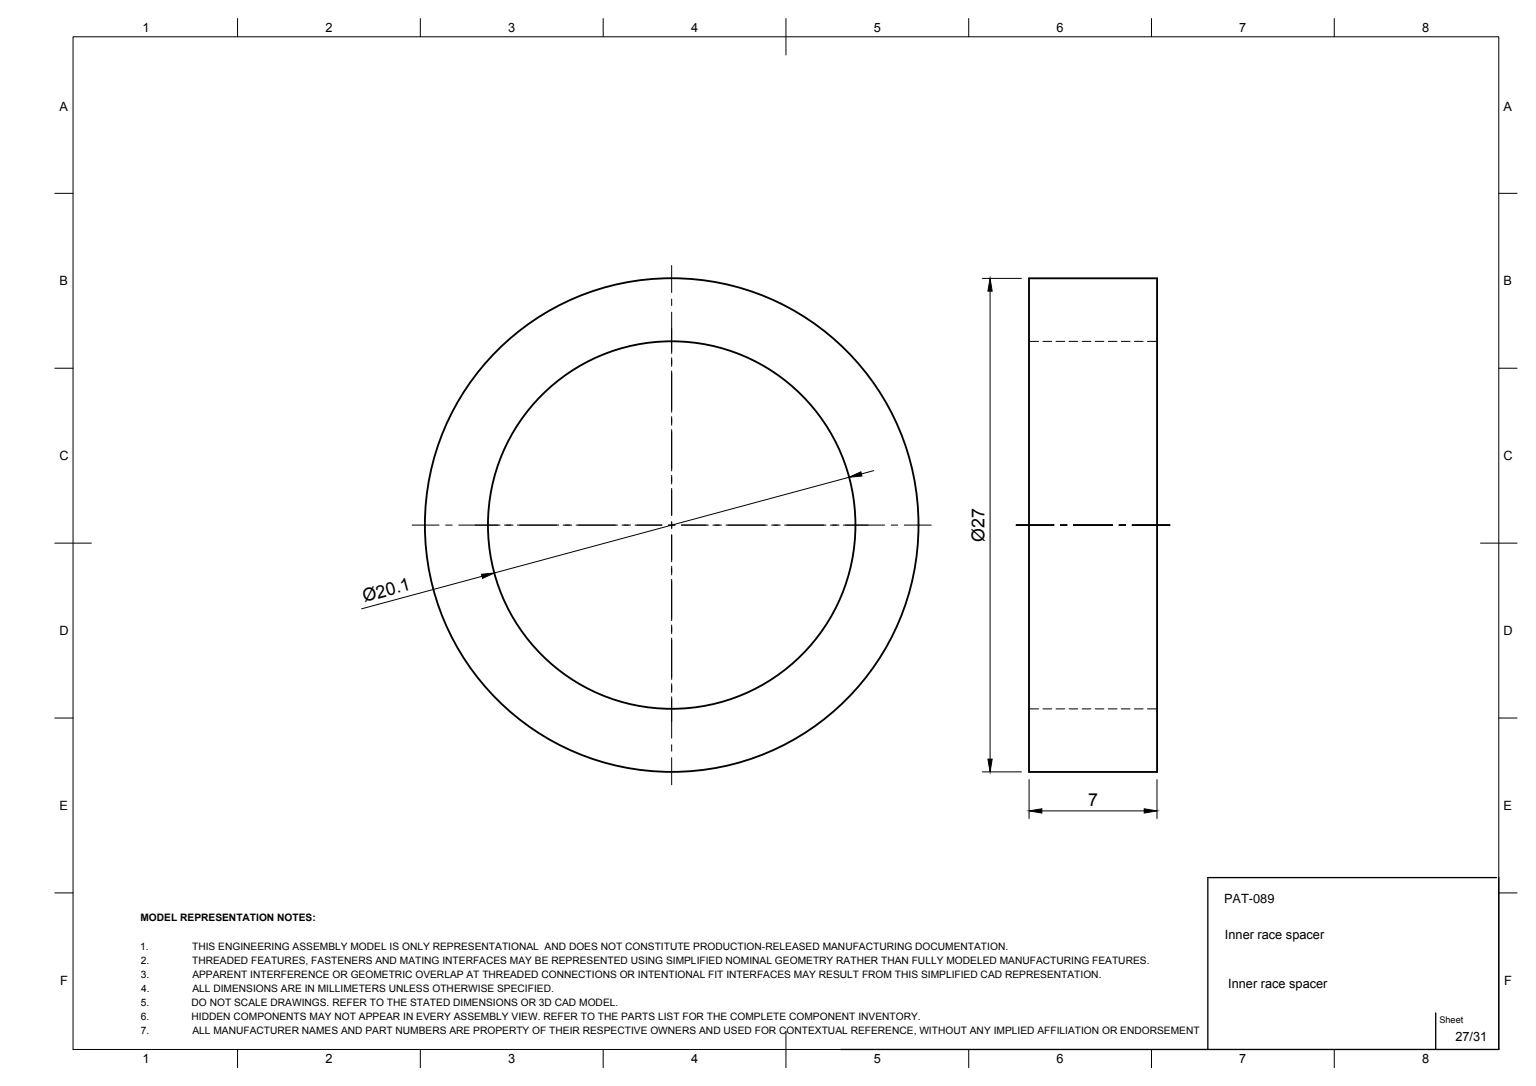
ISO-10303-21;
HEADER;
/* Generated by software containing ST-Developer
 * from STEP Tools, Inc. (www.steptools.com) 
 */

FILE_DESCRIPTION(
/* description */ ('Rotary union on bearing shaft'),
/* implementation_level */ '2;1');

FILE_NAME(
/* name */ 'Inner race spacer.step',
/* time_stamp */ '2026-10-28T03:24:01-07:00',
/* author */ (''),
/* organization */ (''),
/* preprocessor_version */ 'ST-DEVELOPER v20.2',
/* originating_system */ 'Autodesk Translation Framework v15.17.0.0',
/* authorisation */ '');

FILE_SCHEMA (('AUTOMOTIVE_DESIGN { 1 0 10303 214 3 1 1 }'));
ENDSEC;

DATA;
#10=MECHANICAL_DESIGN_GEOMETRIC_PRESENTATION_REPRESENTATION('',(#340),#9448);
#278=SHAPE_REPRESENTATION_RELATIONSHIP('SRR','None',#9580,#305);
#305=ADVANCED_BREP_SHAPE_REPRESENTATION('',(#373),#9440);
#340=STYLED_ITEM('',(#9778),#373);
#373=MANIFOLD_SOLID_BREP('Body1',#4897);
#462=FACE_BOUND('',#1257,.T.);
#463=FACE_BOUND('',#1259,.T.);
#602=PLANE('',#5659);
#603=PLANE('',#5660);
#873=FACE_OUTER_BOUND('',#1254,.T.);
#874=FACE_OUTER_BOUND('',#1255,.T.);
#875=FACE_OUTER_BOUND('',#1256,.T.);
#876=FACE_OUTER_BOUND('',#1258,.T.);
#1254=EDGE_LOOP('',(#4139,#4140,#4141,#4142));
#1255=EDGE_LOOP('',(#4143,#4144,#4145,#4146));
#1256=EDGE_LOOP('',(#4147));
#1257=EDGE_LOOP('',(#4148));
#1258=EDGE_LOOP('',(#4149));
#1259=EDGE_LOOP('',(#4150));
#1564=LINE('',#8922,#1884);
#1565=LINE('',#8928,#1885);
#1884=VECTOR('',#6933,1.005);
#1885=VECTOR('',#6940,1.35);
#2204=CIRCLE('',#5654,1.005);
#2205=CIRCLE('',#5655,1.005);
#2206=CIRCLE('',#5657,1.35);
#2207=CIRCLE('',#5658,1.35);
#2550=VERTEX_POINT('',#8919);
#2551=VERTEX_POINT('',#8921);
#2552=VERTEX_POINT('',#8925);
#2553=VERTEX_POINT('',#8927);
#3097=EDGE_CURVE('',#2550,#2550,#2204,.T.);
#3098=EDGE_CURVE('',#2550,#2551,#1564,.T.);
#3099=EDGE_CURVE('',#2551,#2551,#2205,.T.);
#3100=EDGE_CURVE('',#2552,#2552,#2206,.T.);
#3101=EDGE_CURVE('',#2552,#2553,#1565,.T.);
#3102=EDGE_CURVE('',#2553,#2553,#2207,.T.);
#4139=ORIENTED_EDGE('',*,*,#3097,.F.);
#4140=ORIENTED_EDGE('',*,*,#3098,.T.);
#4141=ORIENTED_EDGE('',*,*,#3099,.T.);
#4142=ORIENTED_EDGE('',*,*,#3098,.F.);
#4143=ORIENTED_EDGE('',*,*,#3100,.F.);
#4144=ORIENTED_EDGE('',*,*,#3101,.T.);
#4145=ORIENTED_EDGE('',*,*,#3102,.T.);
#4146=ORIENTED_EDGE('',*,*,#3101,.F.);
#4147=ORIENTED_EDGE('',*,*,#3100,.T.);
#4148=ORIENTED_EDGE('',*,*,#3097,.T.);
#4149=ORIENTED_EDGE('',*,*,#3102,.F.);
#4150=ORIENTED_EDGE('',*,*,#3099,.F.);
#4549=CYLINDRICAL_SURFACE('',#5653,1.005);
#4550=CYLINDRICAL_SURFACE('',#5656,1.35);
#4786=ADVANCED_FACE('',(#873),#4549,.F.);
#4787=ADVANCED_FACE('',(#874),#4550,.T.);
#4788=ADVANCED_FACE('',(#875,#462),#602,.T.);
#4789=ADVANCED_FACE('',(#876,#463),#603,.F.);
#4897=CLOSED_SHELL('',(#4786,#4787,#4788,#4789));
#5652=AXIS2_PLACEMENT_3D('',#8917,#6927,#6928);
#5653=AXIS2_PLACEMENT_3D('',#8918,#6929,#6930);
#5654=AXIS2_PLACEMENT_3D('',#8920,#6931,#6932);
#5655=AXIS2_PLACEMENT_3D('',#8923,#6934,#6935);
#5656=AXIS2_PLACEMENT_3D('',#8924,#6936,#6937);
#5657=AXIS2_PLACEMENT_3D('',#8926,#6938,#6939);
#5658=AXIS2_PLACEMENT_3D('',#8929,#6941,#6942);
#5659=AXIS2_PLACEMENT_3D('',#8930,#6943,#6944);
#5660=AXIS2_PLACEMENT_3D('',#8931,#6945,#6946);
#6927=DIRECTION('axis',(0.,0.,1.));
#6928=DIRECTION('refdir',(1.,0.,0.));
#6929=DIRECTION('center_axis',(0.,1.,0.));
#6930=DIRECTION('ref_axis',(1.,0.,0.));
#6931=DIRECTION('center_axis',(0.,-1.,0.));
#6932=DIRECTION('ref_axis',(1.,0.,0.));
#6933=DIRECTION('',(0.,-1.,0.));
#6934=DIRECTION('center_axis',(0.,-1.,0.));
#6935=DIRECTION('ref_axis',(1.,0.,0.));
#6936=DIRECTION('center_axis',(0.,1.,0.));
#6937=DIRECTION('ref_axis',(1.,0.,0.));
#6938=DIRECTION('center_axis',(0.,1.,0.));
#6939=DIRECTION('ref_axis',(1.,0.,0.));
#6940=DIRECTION('',(0.,-1.,0.));
#6941=DIRECTION('center_axis',(0.,1.,0.));
#6942=DIRECTION('ref_axis',(1.,0.,0.));
#6943=DIRECTION('center_axis',(0.,1.,0.));
#6944=DIRECTION('ref_axis',(1.,0.,0.));
#6945=DIRECTION('center_axis',(0.,1.,0.));
#6946=DIRECTION('ref_axis',(1.,0.,0.));
#8917=CARTESIAN_POINT('',(0.,0.,0.));
#8918=CARTESIAN_POINT('Origin',(0.,5.7,4.5));
#8919=CARTESIAN_POINT('',(-1.005,6.4,4.5));
#8920=CARTESIAN_POINT('Origin',(0.,6.4,4.5));
#8921=CARTESIAN_POINT('',(-1.005,5.7,4.5));
#8922=CARTESIAN_POINT('',(-1.005,5.7,4.5));
#8923=CARTESIAN_POINT('Origin',(0.,5.7,4.5));
#8924=CARTESIAN_POINT('Origin',(0.,5.7,4.5));
#8925=CARTESIAN_POINT('',(-1.35,6.4,4.5));
#8926=CARTESIAN_POINT('Origin',(0.,6.4,4.5));
#8927=CARTESIAN_POINT('',(-1.35,5.7,4.5));
#8928=CARTESIAN_POINT('',(-1.35,5.7,4.5));
#8929=CARTESIAN_POINT('Origin',(0.,5.7,4.5));
#8930=CARTESIAN_POINT('Origin',(0.,6.4,4.5));
#8931=CARTESIAN_POINT('Origin',(0.,5.7,4.5));
#9408=UNCERTAINTY_MEASURE_WITH_UNIT(LENGTH_MEASURE(0.001),#9449,
'DISTANCE_ACCURACY_VALUE',
'Maximum model space distance between geometric entities at asserted c
onnectivities');
#9416=UNCERTAINTY_MEASURE_WITH_UNIT(LENGTH_MEASURE(0.001),#9449,
'DISTANCE_ACCURACY_VALUE',
'Maximum model space distance between geometric entities at asserted c
onnectivities');
#9440=(
GEOMETRIC_REPRESENTATION_CONTEXT(3)
GLOBAL_UNCERTAINTY_ASSIGNED_CONTEXT((#9408))
GLOBAL_UNIT_ASSIGNED_CONTEXT((#9449,#9451,#9452))
REPRESENTATION_CONTEXT('','3D')
);
#9448=(
GEOMETRIC_REPRESENTATION_CONTEXT(3)
GLOBAL_UNCERTAINTY_ASSIGNED_CONTEXT((#9416))
GLOBAL_UNIT_ASSIGNED_CONTEXT((#9449,#9451,#9452))
REPRESENTATION_CONTEXT('','3D')
);
#9449=(
LENGTH_UNIT()
NAMED_UNIT(*)
SI_UNIT(.CENTI.,.METRE.)
);
#9451=(
NAMED_UNIT(*)
PLANE_ANGLE_UNIT()
SI_UNIT($,.RADIAN.)
);
#9452=(
NAMED_UNIT(*)
SI_UNIT($,.STERADIAN.)
SOLID_ANGLE_UNIT()
);
#9476=SHAPE_DEFINITION_REPRESENTATION(#9512,#9580);
#9512=PRODUCT_DEFINITION_SHAPE('',$,#9612);
#9580=SHAPE_REPRESENTATION('',(#5652),#9440);
#9588=PRODUCT_DEFINITION_CONTEXT('part definition',#9683,'design');
#9612=PRODUCT_DEFINITION('Inner race spacer','Inner race spacer',#9643,
#9588);
#9643=PRODUCT_DEFINITION_FORMATION('',$,#9708);
#9683=APPLICATION_CONTEXT(
'Core Data for Automotive Mechanical Design Process');
#9684=PRODUCT_CONTEXT('part definition',#9683,'mechanical');
#9708=PRODUCT('Inner race spacer','Inner race spacer',
'Inner race spacer',(#9684));
#9772=COLOUR_RGB('Grey',0.48,0.52,0.57);
#9773=FILL_AREA_STYLE_COLOUR('',#9772);
#9774=FILL_AREA_STYLE('',(#9773));
#9775=SURFACE_STYLE_FILL_AREA(#9774);
#9776=SURFACE_SIDE_STYLE('',(#9775));
#9777=SURFACE_STYLE_USAGE(.BOTH.,#9776);
#9778=PRESENTATION_STYLE_ASSIGNMENT((#9777));
ENDSEC;
END-ISO-10303-21;
